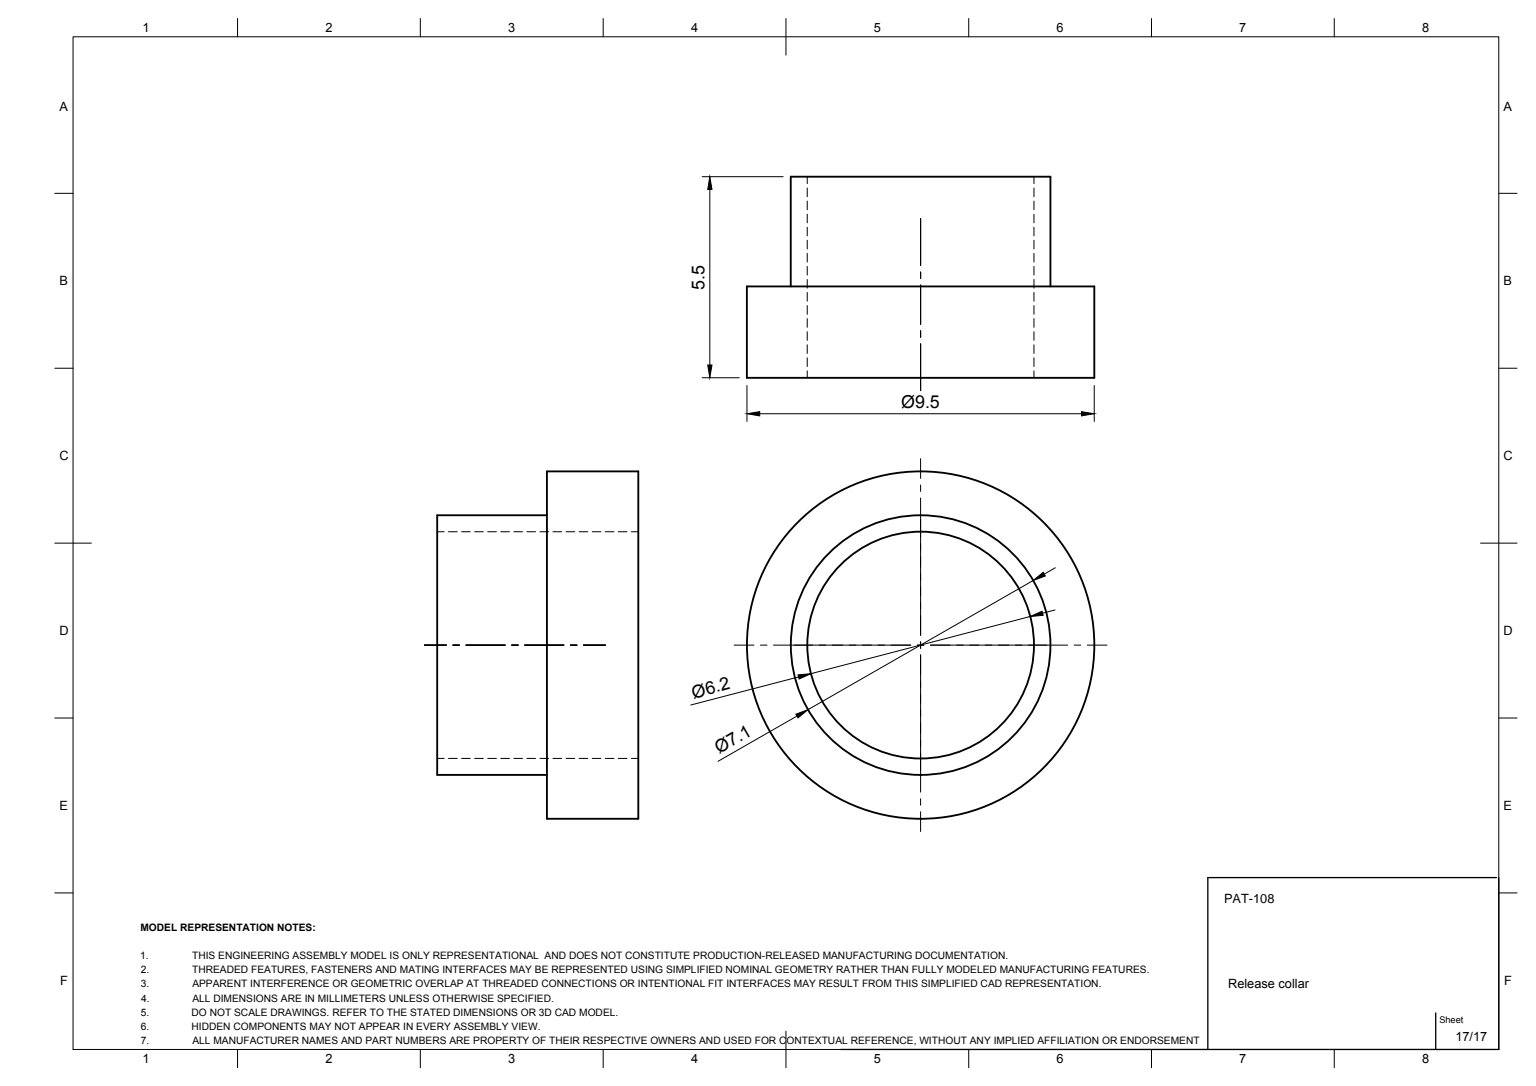
ISO-10303-21;
HEADER;
/* Generated by software containing ST-Developer
 * from STEP Tools, Inc. (www.steptools.com) 
 */

FILE_DESCRIPTION(
/* description */ ('Sub-base valve envelopes and connections'),
/* implementation_level */ '2;1');

FILE_NAME(
/* name */ 'Release collar.step',
/* time_stamp */ '2026-10-29T15:55:44-07:00',
/* author */ (''),
/* organization */ (''),
/* preprocessor_version */ 'ST-DEVELOPER v20.2',
/* originating_system */ 'Autodesk Translation Framework v15.17.0.0',
/* authorisation */ '');

FILE_SCHEMA (('AUTOMOTIVE_DESIGN { 1 0 10303 214 3 1 1 }'));
ENDSEC;

DATA;
#10=MECHANICAL_DESIGN_GEOMETRIC_PRESENTATION_REPRESENTATION('',(#129),#6113);
#105=SHAPE_REPRESENTATION_RELATIONSHIP('SRR','None',#6180,#117);
#117=ADVANCED_BREP_SHAPE_REPRESENTATION('',(#141),#6111);
#129=STYLED_ITEM('',(#6329),#141);
#141=MANIFOLD_SOLID_BREP('Body1',#3368);
#255=FACE_BOUND('',#875,.T.);
#256=FACE_BOUND('',#878,.T.);
#257=FACE_BOUND('',#881,.T.);
#372=PLANE('',#3848);
#373=PLANE('',#3853);
#374=PLANE('',#3857);
#562=FACE_OUTER_BOUND('',#874,.T.);
#563=FACE_OUTER_BOUND('',#876,.T.);
#564=FACE_OUTER_BOUND('',#877,.T.);
#565=FACE_OUTER_BOUND('',#879,.T.);
#566=FACE_OUTER_BOUND('',#880,.T.);
#567=FACE_OUTER_BOUND('',#882,.T.);
#874=EDGE_LOOP('',(#2993));
#875=EDGE_LOOP('',(#2994));
#876=EDGE_LOOP('',(#2995,#2996,#2997,#2998));
#877=EDGE_LOOP('',(#2999));
#878=EDGE_LOOP('',(#3000));
#879=EDGE_LOOP('',(#3001,#3002,#3003,#3004));
#880=EDGE_LOOP('',(#3005));
#881=EDGE_LOOP('',(#3006));
#882=EDGE_LOOP('',(#3007,#3008,#3009,#3010));
#1108=LINE('',#5980,#1342);
#1109=LINE('',#5987,#1343);
#1110=LINE('',#5992,#1344);
#1342=VECTOR('',#4810,0.475);
#1343=VECTOR('',#4819,0.355);
#1344=VECTOR('',#4826,0.31);
#1523=CIRCLE('',#3849,0.475);
#1524=CIRCLE('',#3850,0.31);
#1525=CIRCLE('',#3852,0.475);
#1526=CIRCLE('',#3854,0.355);
#1527=CIRCLE('',#3856,0.355);
#1528=CIRCLE('',#3858,0.31);
#1789=VERTEX_POINT('',#5973);
#1790=VERTEX_POINT('',#5975);
#1791=VERTEX_POINT('',#5978);
#1792=VERTEX_POINT('',#5982);
#1793=VERTEX_POINT('',#5985);
#1794=VERTEX_POINT('',#5989);
#2194=EDGE_CURVE('',#1789,#1789,#1523,.T.);
#2195=EDGE_CURVE('',#1790,#1790,#1524,.T.);
#2196=EDGE_CURVE('',#1791,#1791,#1525,.T.);
#2197=EDGE_CURVE('',#1791,#1789,#1108,.T.);
#2198=EDGE_CURVE('',#1792,#1792,#1526,.T.);
#2199=EDGE_CURVE('',#1793,#1793,#1527,.T.);
#2200=EDGE_CURVE('',#1793,#1792,#1109,.T.);
#2201=EDGE_CURVE('',#1794,#1794,#1528,.T.);
#2202=EDGE_CURVE('',#1794,#1790,#1110,.T.);
#2993=ORIENTED_EDGE('',*,*,#2194,.F.);
#2994=ORIENTED_EDGE('',*,*,#2195,.T.);
#2995=ORIENTED_EDGE('',*,*,#2196,.F.);
#2996=ORIENTED_EDGE('',*,*,#2197,.T.);
#2997=ORIENTED_EDGE('',*,*,#2194,.T.);
#2998=ORIENTED_EDGE('',*,*,#2197,.F.);
#2999=ORIENTED_EDGE('',*,*,#2196,.T.);
#3000=ORIENTED_EDGE('',*,*,#2198,.F.);
#3001=ORIENTED_EDGE('',*,*,#2199,.F.);
#3002=ORIENTED_EDGE('',*,*,#2200,.T.);
#3003=ORIENTED_EDGE('',*,*,#2198,.T.);
#3004=ORIENTED_EDGE('',*,*,#2200,.F.);
#3005=ORIENTED_EDGE('',*,*,#2199,.T.);
#3006=ORIENTED_EDGE('',*,*,#2201,.F.);
#3007=ORIENTED_EDGE('',*,*,#2201,.T.);
#3008=ORIENTED_EDGE('',*,*,#2202,.T.);
#3009=ORIENTED_EDGE('',*,*,#2195,.F.);
#3010=ORIENTED_EDGE('',*,*,#2202,.F.);
#3154=CYLINDRICAL_SURFACE('',#3851,0.475);
#3155=CYLINDRICAL_SURFACE('',#3855,0.355);
#3156=CYLINDRICAL_SURFACE('',#3859,0.31);
#3335=ADVANCED_FACE('',(#562,#255),#372,.T.);
#3336=ADVANCED_FACE('',(#563),#3154,.T.);
#3337=ADVANCED_FACE('',(#564,#256),#373,.T.);
#3338=ADVANCED_FACE('',(#565),#3155,.T.);
#3339=ADVANCED_FACE('',(#566,#257),#374,.T.);
#3340=ADVANCED_FACE('',(#567),#3156,.F.);
#3368=CLOSED_SHELL('',(#3335,#3336,#3337,#3338,#3339,#3340));
#3847=AXIS2_PLACEMENT_3D('',#5971,#4798,#4799);
#3848=AXIS2_PLACEMENT_3D('',#5972,#4800,#4801);
#3849=AXIS2_PLACEMENT_3D('',#5974,#4802,#4803);
#3850=AXIS2_PLACEMENT_3D('',#5976,#4804,#4805);
#3851=AXIS2_PLACEMENT_3D('',#5977,#4806,#4807);
#3852=AXIS2_PLACEMENT_3D('',#5979,#4808,#4809);
#3853=AXIS2_PLACEMENT_3D('',#5981,#4811,#4812);
#3854=AXIS2_PLACEMENT_3D('',#5983,#4813,#4814);
#3855=AXIS2_PLACEMENT_3D('',#5984,#4815,#4816);
#3856=AXIS2_PLACEMENT_3D('',#5986,#4817,#4818);
#3857=AXIS2_PLACEMENT_3D('',#5988,#4820,#4821);
#3858=AXIS2_PLACEMENT_3D('',#5990,#4822,#4823);
#3859=AXIS2_PLACEMENT_3D('',#5991,#4824,#4825);
#4798=DIRECTION('axis',(0.,0.,1.));
#4799=DIRECTION('refdir',(1.,0.,0.));
#4800=DIRECTION('center_axis',(0.,1.,0.));
#4801=DIRECTION('ref_axis',(0.,0.,1.));
#4802=DIRECTION('center_axis',(0.,-1.,0.));
#4803=DIRECTION('ref_axis',(1.,0.,0.));
#4804=DIRECTION('center_axis',(0.,-1.,0.));
#4805=DIRECTION('ref_axis',(1.,0.,0.));
#4806=DIRECTION('center_axis',(0.,-1.,0.));
#4807=DIRECTION('ref_axis',(1.,0.,0.));
#4808=DIRECTION('center_axis',(0.,-1.,0.));
#4809=DIRECTION('ref_axis',(1.,0.,0.));
#4810=DIRECTION('',(0.,1.,0.));
#4811=DIRECTION('center_axis',(0.,-1.,0.));
#4812=DIRECTION('ref_axis',(0.,0.,-1.));
#4813=DIRECTION('center_axis',(0.,-1.,0.));
#4814=DIRECTION('ref_axis',(1.,0.,0.));
#4815=DIRECTION('center_axis',(0.,-1.,0.));
#4816=DIRECTION('ref_axis',(1.,0.,0.));
#4817=DIRECTION('center_axis',(0.,-1.,0.));
#4818=DIRECTION('ref_axis',(1.,0.,0.));
#4819=DIRECTION('',(0.,1.,0.));
#4820=DIRECTION('center_axis',(0.,-1.,0.));
#4821=DIRECTION('ref_axis',(0.,0.,-1.));
#4822=DIRECTION('center_axis',(0.,-1.,0.));
#4823=DIRECTION('ref_axis',(1.,0.,0.));
#4824=DIRECTION('center_axis',(0.,-1.,0.));
#4825=DIRECTION('ref_axis',(1.,0.,0.));
#4826=DIRECTION('',(0.,1.,0.));
#5971=CARTESIAN_POINT('',(0.,0.,0.));
#5972=CARTESIAN_POINT('Origin',(0.475,1.95,0.));
#5973=CARTESIAN_POINT('',(-0.475,1.95,-5.81707229594993E-17));
#5974=CARTESIAN_POINT('Origin',(0.,1.95,0.));
#5975=CARTESIAN_POINT('',(-0.31,1.95,-3.7964050773568E-17));
#5976=CARTESIAN_POINT('Origin',(0.,1.95,0.));
#5977=CARTESIAN_POINT('Origin',(0.,1.825,0.));
#5978=CARTESIAN_POINT('',(-0.475,1.7,-5.81707229594993E-17));
#5979=CARTESIAN_POINT('Origin',(0.,1.7,0.));
#5980=CARTESIAN_POINT('',(-0.475,1.825,-5.81707229594993E-17));
#5981=CARTESIAN_POINT('Origin',(0.355,1.7,0.));
#5982=CARTESIAN_POINT('',(-0.355,1.7,-4.3474961369731E-17));
#5983=CARTESIAN_POINT('Origin',(0.,1.7,0.));
#5984=CARTESIAN_POINT('Origin',(0.,1.55,0.));
#5985=CARTESIAN_POINT('',(-0.355,1.4,-4.3474961369731E-17));
#5986=CARTESIAN_POINT('Origin',(0.,1.4,0.));
#5987=CARTESIAN_POINT('',(-0.355,1.55,-4.3474961369731E-17));
#5988=CARTESIAN_POINT('Origin',(0.31,1.4,0.));
#5989=CARTESIAN_POINT('',(-0.31,1.4,-3.7964050773568E-17));
#5990=CARTESIAN_POINT('Origin',(0.,1.4,0.));
#5991=CARTESIAN_POINT('Origin',(0.,1.675,0.));
#5992=CARTESIAN_POINT('',(-0.31,1.675,-3.7964050773568E-17));
#6095=UNCERTAINTY_MEASURE_WITH_UNIT(LENGTH_MEASURE(0.001),#6114,
'DISTANCE_ACCURACY_VALUE',
'Maximum model space distance between geometric entities at asserted c
onnectivities');
#6097=UNCERTAINTY_MEASURE_WITH_UNIT(LENGTH_MEASURE(0.001),#6114,
'DISTANCE_ACCURACY_VALUE',
'Maximum model space distance between geometric entities at asserted c
onnectivities');
#6111=(
GEOMETRIC_REPRESENTATION_CONTEXT(3)
GLOBAL_UNCERTAINTY_ASSIGNED_CONTEXT((#6095))
GLOBAL_UNIT_ASSIGNED_CONTEXT((#6114,#6116,#6117))
REPRESENTATION_CONTEXT('','3D')
);
#6113=(
GEOMETRIC_REPRESENTATION_CONTEXT(3)
GLOBAL_UNCERTAINTY_ASSIGNED_CONTEXT((#6097))
GLOBAL_UNIT_ASSIGNED_CONTEXT((#6114,#6116,#6117))
REPRESENTATION_CONTEXT('','3D')
);
#6114=(
LENGTH_UNIT()
NAMED_UNIT(*)
SI_UNIT(.CENTI.,.METRE.)
);
#6116=(
NAMED_UNIT(*)
PLANE_ANGLE_UNIT()
SI_UNIT($,.RADIAN.)
);
#6117=(
NAMED_UNIT(*)
SI_UNIT($,.STERADIAN.)
SOLID_ANGLE_UNIT()
);
#6131=SHAPE_DEFINITION_REPRESENTATION(#6146,#6180);
#6146=PRODUCT_DEFINITION_SHAPE('',$,#6196);
#6180=SHAPE_REPRESENTATION('',(#3847),#6111);
#6182=PRODUCT_DEFINITION_CONTEXT('part definition',#6229,'design');
#6196=PRODUCT_DEFINITION('Release collar','Release collar',#6211,
#6182);
#6211=PRODUCT_DEFINITION_FORMATION('',$,#6244);
#6229=APPLICATION_CONTEXT(
'Core Data for Automotive Mechanical Design Process');
#6230=PRODUCT_CONTEXT('part definition',#6229,'mechanical');
#6244=PRODUCT('Release collar','Release collar',
'Release collar',(#6230));
#6323=COLOUR_RGB('Off White',0.89,0.88,0.83);
#6324=FILL_AREA_STYLE_COLOUR('',#6323);
#6325=FILL_AREA_STYLE('',(#6324));
#6326=SURFACE_STYLE_FILL_AREA(#6325);
#6327=SURFACE_SIDE_STYLE('',(#6326));
#6328=SURFACE_STYLE_USAGE(.BOTH.,#6327);
#6329=PRESENTATION_STYLE_ASSIGNMENT((#6328));
ENDSEC;
END-ISO-10303-21;
